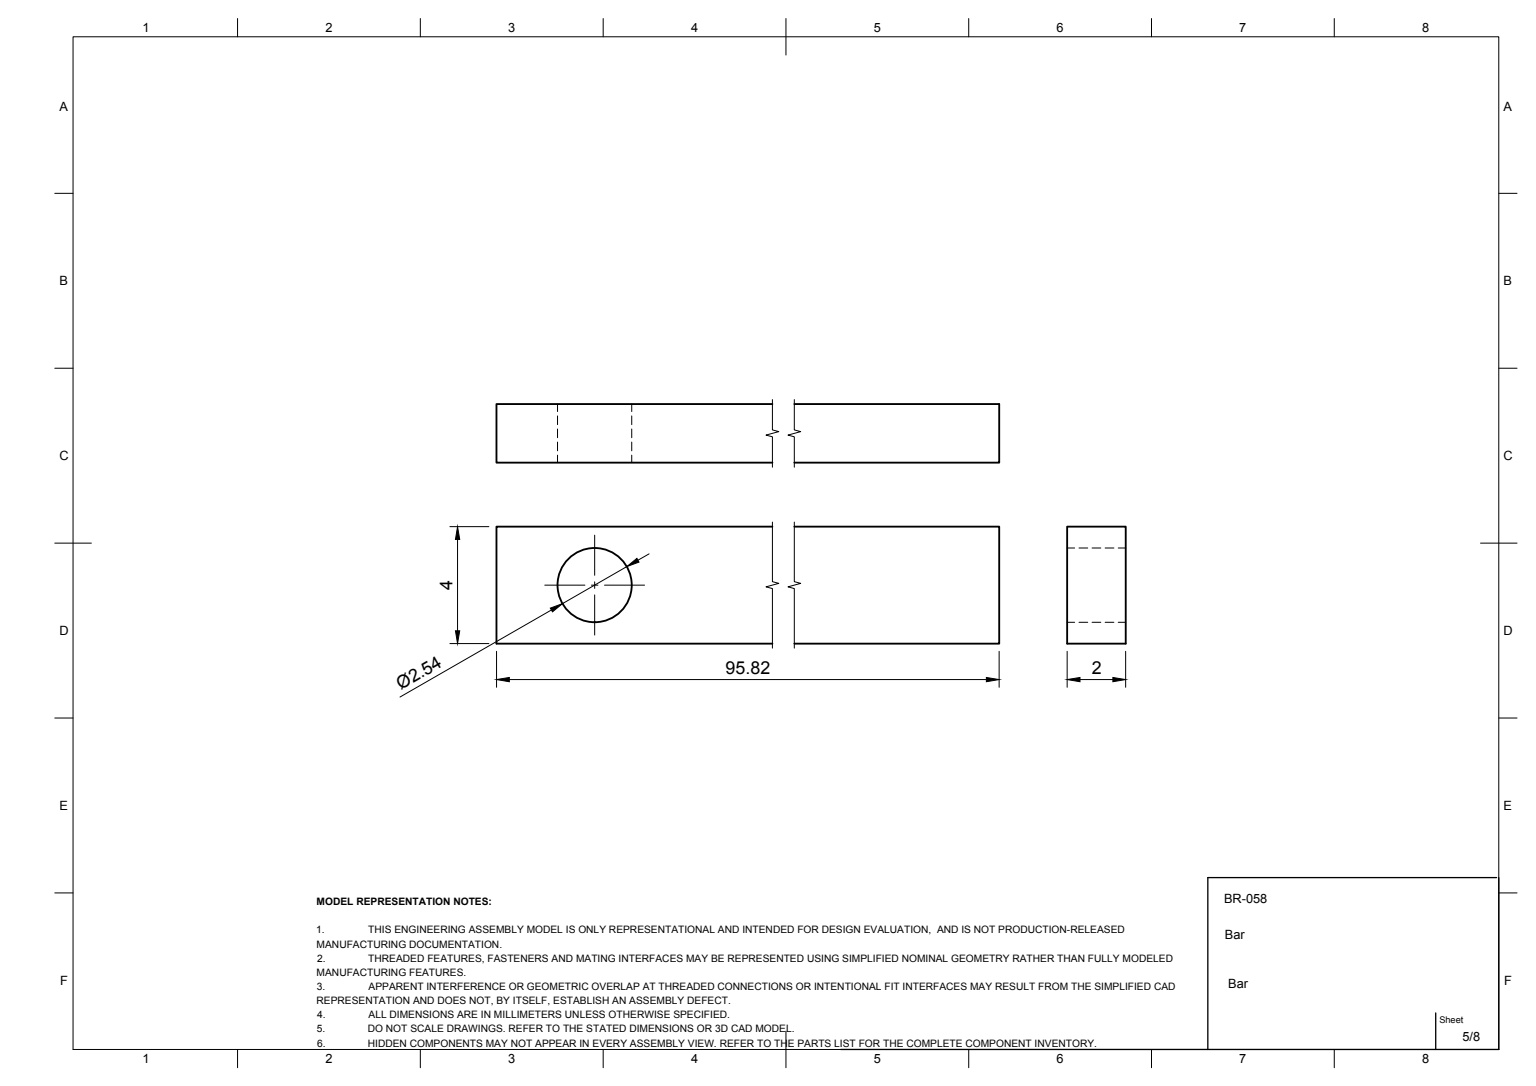
ISO-10303-21;
HEADER;
/* Generated by software containing ST-Developer
 * from STEP Tools, Inc. (www.steptools.com) 
 */

FILE_DESCRIPTION(
/* description */ (''),
/* implementation_level */ '2;1');

FILE_NAME(
/* name */ 'Bar.step',
/* time_stamp */ '2026-10-12T16:07:47-07:00',
/* author */ (''),
/* organization */ (''),
/* preprocessor_version */ 'ST-DEVELOPER v20.2',
/* originating_system */ 'Autodesk Translation Framework v15.15.0.0',
/* authorisation */ '');

FILE_SCHEMA (('AUTOMOTIVE_DESIGN { 1 0 10303 214 3 1 1 }'));
ENDSEC;

DATA;
#10=MECHANICAL_DESIGN_GEOMETRIC_PRESENTATION_REPRESENTATION('',(#95),#8779);
#81=SHAPE_REPRESENTATION_RELATIONSHIP('SRR','None',#8810,#88);
#88=ADVANCED_BREP_SHAPE_REPRESENTATION('',(#105),#8773);
#95=STYLED_ITEM('',(#8854),#105);
#105=MANIFOLD_SOLID_BREP('Body1',#5115);
#146=FACE_BOUND('',#973,.T.);
#147=FACE_BOUND('',#975,.T.);
#291=CIRCLE('',#5511,1.26938918348039);
#292=CIRCLE('',#5512,1.26938918348039);
#457=CYLINDRICAL_SURFACE('',#5510,1.26938918348039);
#658=FACE_OUTER_BOUND('',#967,.T.);
#659=FACE_OUTER_BOUND('',#968,.T.);
#660=FACE_OUTER_BOUND('',#969,.T.);
#661=FACE_OUTER_BOUND('',#970,.T.);
#662=FACE_OUTER_BOUND('',#971,.T.);
#663=FACE_OUTER_BOUND('',#972,.T.);
#664=FACE_OUTER_BOUND('',#974,.T.);
#967=EDGE_LOOP('',(#4326,#4327,#4328,#4329));
#968=EDGE_LOOP('',(#4330,#4331,#4332,#4333));
#969=EDGE_LOOP('',(#4334,#4335,#4336,#4337));
#970=EDGE_LOOP('',(#4338,#4339,#4340,#4341));
#971=EDGE_LOOP('',(#4342,#4343,#4344,#4345));
#972=EDGE_LOOP('',(#4346,#4347,#4348,#4349));
#973=EDGE_LOOP('',(#4350));
#974=EDGE_LOOP('',(#4351,#4352,#4353,#4354));
#975=EDGE_LOOP('',(#4355));
#1505=LINE('',#8342,#1990);
#1506=LINE('',#8347,#1991);
#1507=LINE('',#8349,#1992);
#1508=LINE('',#8351,#1993);
#1509=LINE('',#8352,#1994);
#1510=LINE('',#8355,#1995);
#1511=LINE('',#8357,#1996);
#1512=LINE('',#8358,#1997);
#1513=LINE('',#8361,#1998);
#1514=LINE('',#8363,#1999);
#1515=LINE('',#8364,#2000);
#1516=LINE('',#8366,#2001);
#1517=LINE('',#8367,#2002);
#1990=VECTOR('',#6763,1.26938918348039);
#1991=VECTOR('',#6768,10.);
#1992=VECTOR('',#6769,10.);
#1993=VECTOR('',#6770,10.);
#1994=VECTOR('',#6771,10.);
#1995=VECTOR('',#6774,10.);
#1996=VECTOR('',#6775,10.);
#1997=VECTOR('',#6776,10.);
#1998=VECTOR('',#6779,10.);
#1999=VECTOR('',#6780,10.);
#2000=VECTOR('',#6781,10.);
#2001=VECTOR('',#6784,10.);
#2002=VECTOR('',#6785,10.);
#2416=VERTEX_POINT('',#8339);
#2417=VERTEX_POINT('',#8341);
#2418=VERTEX_POINT('',#8345);
#2419=VERTEX_POINT('',#8346);
#2420=VERTEX_POINT('',#8348);
#2421=VERTEX_POINT('',#8350);
#2422=VERTEX_POINT('',#8354);
#2423=VERTEX_POINT('',#8356);
#2424=VERTEX_POINT('',#8360);
#2425=VERTEX_POINT('',#8362);
#3067=EDGE_CURVE('',#2416,#2416,#291,.T.);
#3068=EDGE_CURVE('',#2416,#2417,#1505,.T.);
#3069=EDGE_CURVE('',#2417,#2417,#292,.T.);
#3070=EDGE_CURVE('',#2418,#2419,#1506,.T.);
#3071=EDGE_CURVE('',#2419,#2420,#1507,.T.);
#3072=EDGE_CURVE('',#2420,#2421,#1508,.T.);
#3073=EDGE_CURVE('',#2418,#2421,#1509,.T.);
#3074=EDGE_CURVE('',#2418,#2422,#1510,.T.);
#3075=EDGE_CURVE('',#2423,#2421,#1511,.T.);
#3076=EDGE_CURVE('',#2422,#2423,#1512,.T.);
#3077=EDGE_CURVE('',#2422,#2424,#1513,.T.);
#3078=EDGE_CURVE('',#2425,#2423,#1514,.T.);
#3079=EDGE_CURVE('',#2424,#2425,#1515,.T.);
#3080=EDGE_CURVE('',#2424,#2419,#1516,.T.);
#3081=EDGE_CURVE('',#2425,#2420,#1517,.T.);
#4326=ORIENTED_EDGE('',*,*,#3067,.F.);
#4327=ORIENTED_EDGE('',*,*,#3068,.T.);
#4328=ORIENTED_EDGE('',*,*,#3069,.F.);
#4329=ORIENTED_EDGE('',*,*,#3068,.F.);
#4330=ORIENTED_EDGE('',*,*,#3070,.T.);
#4331=ORIENTED_EDGE('',*,*,#3071,.T.);
#4332=ORIENTED_EDGE('',*,*,#3072,.T.);
#4333=ORIENTED_EDGE('',*,*,#3073,.F.);
#4334=ORIENTED_EDGE('',*,*,#3074,.F.);
#4335=ORIENTED_EDGE('',*,*,#3073,.T.);
#4336=ORIENTED_EDGE('',*,*,#3075,.F.);
#4337=ORIENTED_EDGE('',*,*,#3076,.F.);
#4338=ORIENTED_EDGE('',*,*,#3077,.F.);
#4339=ORIENTED_EDGE('',*,*,#3076,.T.);
#4340=ORIENTED_EDGE('',*,*,#3078,.F.);
#4341=ORIENTED_EDGE('',*,*,#3079,.F.);
#4342=ORIENTED_EDGE('',*,*,#3080,.F.);
#4343=ORIENTED_EDGE('',*,*,#3079,.T.);
#4344=ORIENTED_EDGE('',*,*,#3081,.T.);
#4345=ORIENTED_EDGE('',*,*,#3071,.F.);
#4346=ORIENTED_EDGE('',*,*,#3081,.F.);
#4347=ORIENTED_EDGE('',*,*,#3078,.T.);
#4348=ORIENTED_EDGE('',*,*,#3075,.T.);
#4349=ORIENTED_EDGE('',*,*,#3072,.F.);
#4350=ORIENTED_EDGE('',*,*,#3067,.T.);
#4351=ORIENTED_EDGE('',*,*,#3080,.T.);
#4352=ORIENTED_EDGE('',*,*,#3070,.F.);
#4353=ORIENTED_EDGE('',*,*,#3074,.T.);
#4354=ORIENTED_EDGE('',*,*,#3077,.T.);
#4355=ORIENTED_EDGE('',*,*,#3069,.T.);
#4794=PLANE('',#5513);
#4795=PLANE('',#5514);
#4796=PLANE('',#5515);
#4797=PLANE('',#5516);
#4798=PLANE('',#5517);
#4799=PLANE('',#5518);
#5020=ADVANCED_FACE('',(#658),#457,.F.);
#5021=ADVANCED_FACE('',(#659),#4794,.F.);
#5022=ADVANCED_FACE('',(#660),#4795,.T.);
#5023=ADVANCED_FACE('',(#661),#4796,.T.);
#5024=ADVANCED_FACE('',(#662),#4797,.T.);
#5025=ADVANCED_FACE('',(#663,#146),#4798,.T.);
#5026=ADVANCED_FACE('',(#664,#147),#4799,.F.);
#5115=CLOSED_SHELL('',(#5020,#5021,#5022,#5023,#5024,#5025,#5026));
#5509=AXIS2_PLACEMENT_3D('',#8337,#6757,#6758);
#5510=AXIS2_PLACEMENT_3D('',#8338,#6759,#6760);
#5511=AXIS2_PLACEMENT_3D('',#8340,#6761,#6762);
#5512=AXIS2_PLACEMENT_3D('',#8343,#6764,#6765);
#5513=AXIS2_PLACEMENT_3D('',#8344,#6766,#6767);
#5514=AXIS2_PLACEMENT_3D('',#8353,#6772,#6773);
#5515=AXIS2_PLACEMENT_3D('',#8359,#6777,#6778);
#5516=AXIS2_PLACEMENT_3D('',#8365,#6782,#6783);
#5517=AXIS2_PLACEMENT_3D('',#8368,#6786,#6787);
#5518=AXIS2_PLACEMENT_3D('',#8369,#6788,#6789);
#6757=DIRECTION('axis',(0.,0.,1.));
#6758=DIRECTION('refdir',(1.,0.,0.));
#6759=DIRECTION('center_axis',(0.,-1.,0.));
#6760=DIRECTION('ref_axis',(1.,0.,0.));
#6761=DIRECTION('center_axis',(0.,-1.,0.));
#6762=DIRECTION('ref_axis',(1.,0.,0.));
#6763=DIRECTION('',(0.,-1.,0.));
#6764=DIRECTION('center_axis',(0.,1.,0.));
#6765=DIRECTION('ref_axis',(1.,0.,0.));
#6766=DIRECTION('center_axis',(1.,0.,0.));
#6767=DIRECTION('ref_axis',(0.,0.,-1.));
#6768=DIRECTION('',(0.,0.,1.));
#6769=DIRECTION('',(0.,1.,0.));
#6770=DIRECTION('',(0.,0.,-1.));
#6771=DIRECTION('',(0.,1.,0.));
#6772=DIRECTION('center_axis',(0.,0.,-1.));
#6773=DIRECTION('ref_axis',(-1.,0.,0.));
#6774=DIRECTION('',(1.,0.,0.));
#6775=DIRECTION('',(-1.,0.,0.));
#6776=DIRECTION('',(0.,1.,0.));
#6777=DIRECTION('center_axis',(1.,0.,0.));
#6778=DIRECTION('ref_axis',(0.,0.,-1.));
#6779=DIRECTION('',(0.,0.,1.));
#6780=DIRECTION('',(0.,0.,-1.));
#6781=DIRECTION('',(0.,1.,0.));
#6782=DIRECTION('center_axis',(0.,0.,1.));
#6783=DIRECTION('ref_axis',(1.,0.,0.));
#6784=DIRECTION('',(-1.,0.,0.));
#6785=DIRECTION('',(-1.,0.,0.));
#6786=DIRECTION('center_axis',(0.,1.,0.));
#6787=DIRECTION('ref_axis',(0.,0.,1.));
#6788=DIRECTION('center_axis',(0.,1.,0.));
#6789=DIRECTION('ref_axis',(1.,0.,0.));
#8337=CARTESIAN_POINT('',(0.,0.,0.));
#8338=CARTESIAN_POINT('Origin',(0.,2.,92.461739559435));
#8339=CARTESIAN_POINT('',(-1.26938918348039,4.,92.461739559435));
#8340=CARTESIAN_POINT('Origin',(0.,4.,92.461739559435));
#8341=CARTESIAN_POINT('',(-1.26938918348039,2.,92.461739559435));
#8342=CARTESIAN_POINT('',(-1.26938918348039,2.,92.461739559435));
#8343=CARTESIAN_POINT('Origin',(0.,2.,92.461739559435));
#8344=CARTESIAN_POINT('Origin',(-2.,2.,95.8170335569158));
#8345=CARTESIAN_POINT('',(-2.,2.,0.));
#8346=CARTESIAN_POINT('',(-2.,2.,95.8170335569158));
#8347=CARTESIAN_POINT('',(-2.,2.,0.));
#8348=CARTESIAN_POINT('',(-2.,4.,95.8170335569158));
#8349=CARTESIAN_POINT('',(-2.,2.,95.8170335569158));
#8350=CARTESIAN_POINT('',(-2.,4.,0.));
#8351=CARTESIAN_POINT('',(-2.,4.,0.));
#8352=CARTESIAN_POINT('',(-2.,2.,0.));
#8353=CARTESIAN_POINT('Origin',(2.,2.,0.));
#8354=CARTESIAN_POINT('',(2.,2.,0.));
#8355=CARTESIAN_POINT('',(0.,2.,0.));
#8356=CARTESIAN_POINT('',(2.,4.,0.));
#8357=CARTESIAN_POINT('',(0.,4.,0.));
#8358=CARTESIAN_POINT('',(2.,2.,0.));
#8359=CARTESIAN_POINT('Origin',(2.,2.,95.8170335569158));
#8360=CARTESIAN_POINT('',(2.,2.,95.8170335569158));
#8361=CARTESIAN_POINT('',(2.,2.,0.));
#8362=CARTESIAN_POINT('',(2.,4.,95.8170335569158));
#8363=CARTESIAN_POINT('',(2.,4.,0.));
#8364=CARTESIAN_POINT('',(2.,2.,95.8170335569158));
#8365=CARTESIAN_POINT('Origin',(0.,2.,95.8170335569158));
#8366=CARTESIAN_POINT('',(2.,2.,95.8170335569158));
#8367=CARTESIAN_POINT('',(-2.,4.,95.8170335569158));
#8368=CARTESIAN_POINT('Origin',(1.,4.,47.9085167784579));
#8369=CARTESIAN_POINT('Origin',(1.,2.,47.9085167784579));
#8764=UNCERTAINTY_MEASURE_WITH_UNIT(LENGTH_MEASURE(0.01),#8780,
'DISTANCE_ACCURACY_VALUE',
'Maximum model space distance between geometric entities at asserted c
onnectivities');
#8770=UNCERTAINTY_MEASURE_WITH_UNIT(LENGTH_MEASURE(0.01),#8780,
'DISTANCE_ACCURACY_VALUE',
'Maximum model space distance between geometric entities at asserted c
onnectivities');
#8773=(
GEOMETRIC_REPRESENTATION_CONTEXT(3)
GLOBAL_UNCERTAINTY_ASSIGNED_CONTEXT((#8764))
GLOBAL_UNIT_ASSIGNED_CONTEXT((#8780,#8782,#8783))
REPRESENTATION_CONTEXT('','3D')
);
#8779=(
GEOMETRIC_REPRESENTATION_CONTEXT(3)
GLOBAL_UNCERTAINTY_ASSIGNED_CONTEXT((#8770))
GLOBAL_UNIT_ASSIGNED_CONTEXT((#8780,#8782,#8783))
REPRESENTATION_CONTEXT('','3D')
);
#8780=(
LENGTH_UNIT()
NAMED_UNIT(*)
SI_UNIT(.MILLI.,.METRE.)
);
#8782=(
NAMED_UNIT(*)
PLANE_ANGLE_UNIT()
SI_UNIT($,.RADIAN.)
);
#8783=(
NAMED_UNIT(*)
SI_UNIT($,.STERADIAN.)
SOLID_ANGLE_UNIT()
);
#8786=SHAPE_DEFINITION_REPRESENTATION(#8794,#8810);
#8794=PRODUCT_DEFINITION_SHAPE('',$,#8819);
#8810=SHAPE_REPRESENTATION('',(#5509),#8773);
#8816=PRODUCT_DEFINITION_CONTEXT('part definition',#8842,'design');
#8819=PRODUCT_DEFINITION('Bar','Bar',#8827,#8816);
#8827=PRODUCT_DEFINITION_FORMATION('',$,#8846);
#8842=APPLICATION_CONTEXT(
'Core Data for Automotive Mechanical Design Process');
#8843=PRODUCT_CONTEXT('part definition',#8842,'mechanical');
#8846=PRODUCT('Bar','Bar',$,(#8843));
#8854=PRESENTATION_STYLE_ASSIGNMENT((#8859));
#8859=SURFACE_STYLE_USAGE(.BOTH.,#8864);
#8864=SURFACE_SIDE_STYLE('',(#8869));
#8869=SURFACE_STYLE_FILL_AREA(#8874);
#8874=FILL_AREA_STYLE('Opaque(85,170,0)',(#8879));
#8879=FILL_AREA_STYLE_COLOUR('Opaque(85,170,0)',#8884);
#8884=COLOUR_RGB('Opaque(85,170,0)', 0.66274510, 0.83137255, 0.94901961);
ENDSEC;
END-ISO-10303-21;
